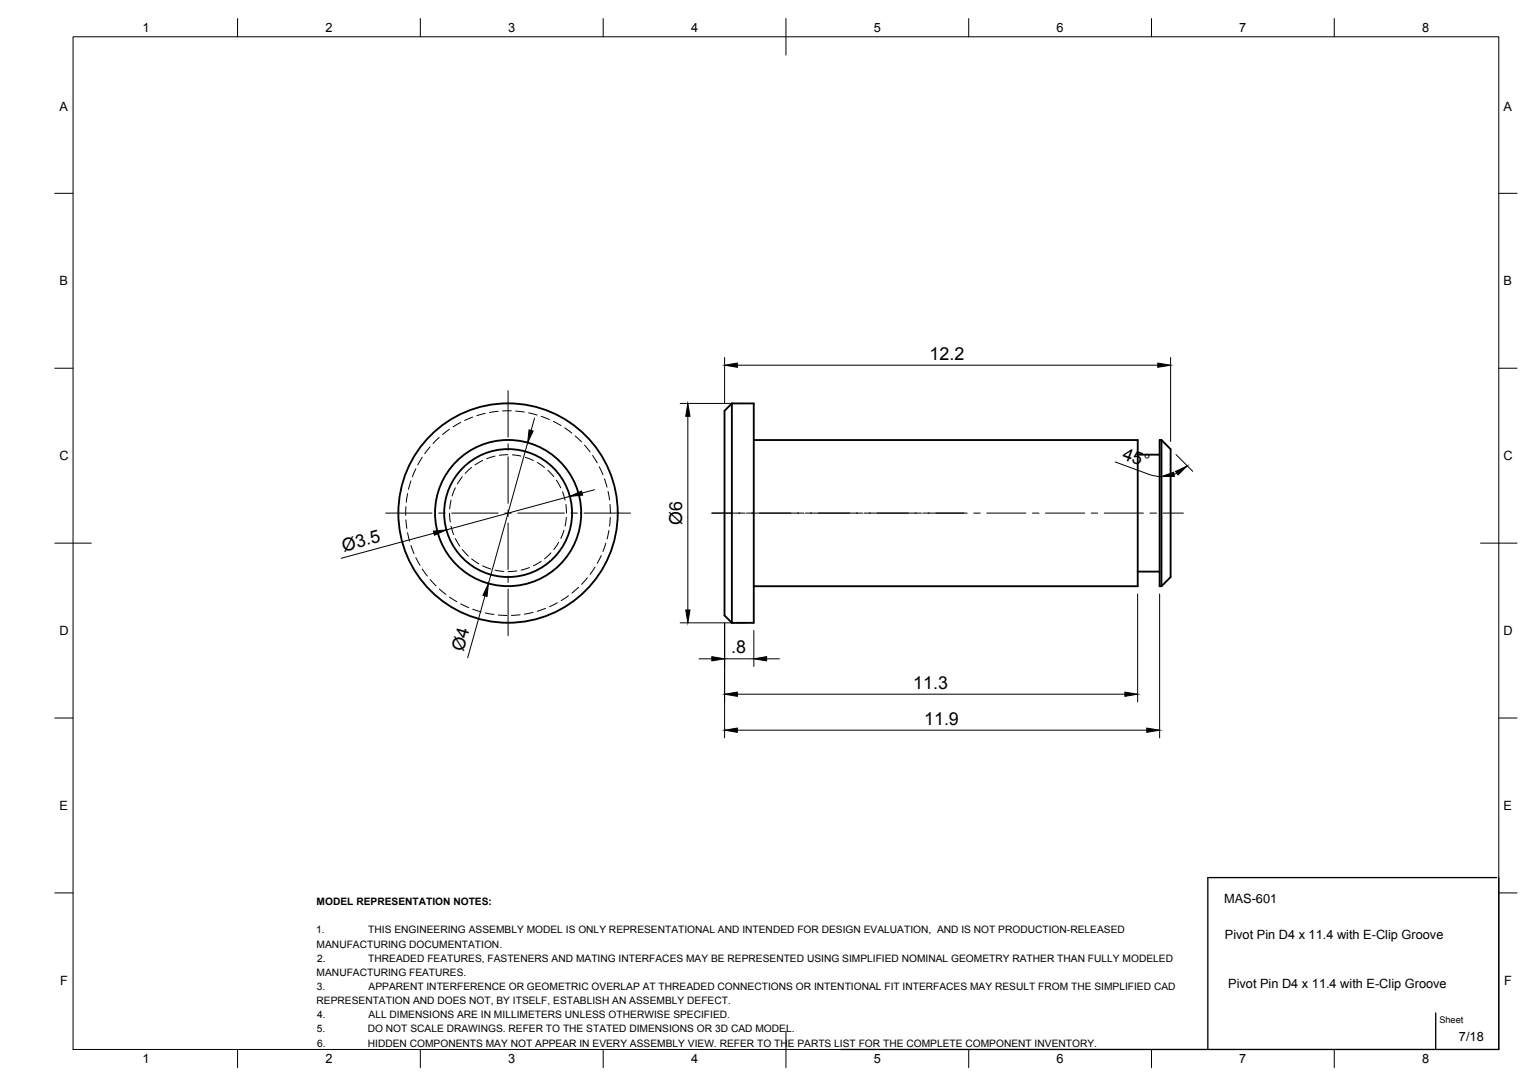
ISO-10303-21;
HEADER;
FILE_DESCRIPTION((''),'2;1');
FILE_NAME('Pivot Pin D4 x 11.4 with E-Clip Groove.step','2026-10-06T07:37:42+05:00',(''),(''),'','','');
FILE_SCHEMA (('AUTOMOTIVE_DESIGN { 1 0 10303 214 3 1 1 }'));
ENDSEC;
DATA;
#10=MECHANICAL_DESIGN_GEOMETRIC_PRESENTATION_REPRESENTATION('',(#383),#18757);
#349=SHAPE_REPRESENTATION_RELATIONSHIP('SRR','None',#18867,#366) ;
#366=ADVANCED_BREP_SHAPE_REPRESENTATION('',(#400),#18750) ;
#383=STYLED_ITEM('',(#18961),#400) ;
#400=MANIFOLD_SOLID_BREP('Pivot Pin D4 x 11.4 with E-Clip Groove',#9552) ;
#588=CYLINDRICAL_SURFACE('',#10224,3.) ;
#589=CYLINDRICAL_SURFACE('',#10228,2.) ;
#590=CYLINDRICAL_SURFACE('',#10232,1.59999999999999) ;
#591=CYLINDRICAL_SURFACE('',#10236,2.) ;
#729=FACE_BOUND('',#1946,.T.) ;
#730=FACE_BOUND('',#1949,.T.) ;
#731=FACE_BOUND('',#1952,.T.) ;
#906=PLANE('',#10220) ;
#907=PLANE('',#10226) ;
#908=PLANE('',#10230) ;
#909=PLANE('',#10234) ;
#910=PLANE('',#10240) ;
#1345=FACE_OUTER_BOUND('',#1942,.T.) ;
#1346=FACE_OUTER_BOUND('',#1943,.T.) ;
#1347=FACE_OUTER_BOUND('',#1944,.T.) ;
#1348=FACE_OUTER_BOUND('',#1945,.T.) ;
#1349=FACE_OUTER_BOUND('',#1947,.T.) ;
#1350=FACE_OUTER_BOUND('',#1948,.T.) ;
#1351=FACE_OUTER_BOUND('',#1950,.T.) ;
#1352=FACE_OUTER_BOUND('',#1951,.T.) ;
#1353=FACE_OUTER_BOUND('',#1953,.T.) ;
#1354=FACE_OUTER_BOUND('',#1954,.T.) ;
#1355=FACE_OUTER_BOUND('',#1955,.T.) ;
#1942=EDGE_LOOP('',(#7637)) ;
#1943=EDGE_LOOP('',(#7638,#7639,#7640,#7641)) ;
#1944=EDGE_LOOP('',(#7642,#7643,#7644,#7645)) ;
#1945=EDGE_LOOP('',(#7646)) ;
#1946=EDGE_LOOP('',(#7647)) ;
#1947=EDGE_LOOP('',(#7648,#7649,#7650,#7651)) ;
#1948=EDGE_LOOP('',(#7652)) ;
#1949=EDGE_LOOP('',(#7653)) ;
#1950=EDGE_LOOP('',(#7654,#7655,#7656,#7657)) ;
#1951=EDGE_LOOP('',(#7658)) ;
#1952=EDGE_LOOP('',(#7659)) ;
#1953=EDGE_LOOP('',(#7660,#7661,#7662,#7663)) ;
#1954=EDGE_LOOP('',(#7664,#7665,#7666,#7667)) ;
#1955=EDGE_LOOP('',(#7668)) ;
#2646=LINE('',#15200,#3417) ;
#2647=LINE('',#15204,#3418) ;
#2648=LINE('',#15211,#3419) ;
#2649=LINE('',#15218,#3420) ;
#2650=LINE('',#15225,#3421) ;
#2651=LINE('',#15229,#3422) ;
#3417=VECTOR('',#12082,2.9) ;
#3418=VECTOR('',#12087,3.) ;
#3419=VECTOR('',#12096,2.) ;
#3420=VECTOR('',#12105,1.59999999999999) ;
#3421=VECTOR('',#12114,2.) ;
#3422=VECTOR('',#12119,1.875) ;
#3978=CIRCLE('',#10221,2.79999999999999) ;
#3979=CIRCLE('',#10223,3.) ;
#3980=CIRCLE('',#10225,3.) ;
#3981=CIRCLE('',#10227,2.) ;
#3982=CIRCLE('',#10229,2.) ;
#3983=CIRCLE('',#10231,1.59999999999999) ;
#3984=CIRCLE('',#10233,1.59999999999999) ;
#3985=CIRCLE('',#10235,2.) ;
#3986=CIRCLE('',#10237,2.) ;
#3987=CIRCLE('',#10239,1.75) ;
#4575=VERTEX_POINT('',#15195) ;
#4576=VERTEX_POINT('',#15198) ;
#4577=VERTEX_POINT('',#15202) ;
#4578=VERTEX_POINT('',#15206) ;
#4579=VERTEX_POINT('',#15209) ;
#4580=VERTEX_POINT('',#15213) ;
#4581=VERTEX_POINT('',#15216) ;
#4582=VERTEX_POINT('',#15220) ;
#4583=VERTEX_POINT('',#15223) ;
#4584=VERTEX_POINT('',#15227) ;
#5665=EDGE_CURVE('',#4575,#4575,#3978,.T.) ;
#5666=EDGE_CURVE('',#4576,#4576,#3979,.T.) ;
#5667=EDGE_CURVE('',#4576,#4575,#2646,.T.) ;
#5668=EDGE_CURVE('',#4577,#4577,#3980,.T.) ;
#5669=EDGE_CURVE('',#4577,#4576,#2647,.T.) ;
#5670=EDGE_CURVE('',#4578,#4578,#3981,.T.) ;
#5671=EDGE_CURVE('',#4579,#4579,#3982,.T.) ;
#5672=EDGE_CURVE('',#4579,#4578,#2648,.T.) ;
#5673=EDGE_CURVE('',#4580,#4580,#3983,.T.) ;
#5674=EDGE_CURVE('',#4581,#4581,#3984,.T.) ;
#5675=EDGE_CURVE('',#4581,#4580,#2649,.T.) ;
#5676=EDGE_CURVE('',#4582,#4582,#3985,.T.) ;
#5677=EDGE_CURVE('',#4583,#4583,#3986,.T.) ;
#5678=EDGE_CURVE('',#4583,#4582,#2650,.T.) ;
#5679=EDGE_CURVE('',#4584,#4584,#3987,.T.) ;
#5680=EDGE_CURVE('',#4584,#4583,#2651,.T.) ;
#7637=ORIENTED_EDGE('',*,*,#5665,.F.) ;
#7638=ORIENTED_EDGE('',*,*,#5666,.F.) ;
#7639=ORIENTED_EDGE('',*,*,#5667,.T.) ;
#7640=ORIENTED_EDGE('',*,*,#5665,.T.) ;
#7641=ORIENTED_EDGE('',*,*,#5667,.F.) ;
#7642=ORIENTED_EDGE('',*,*,#5668,.F.) ;
#7643=ORIENTED_EDGE('',*,*,#5669,.T.) ;
#7644=ORIENTED_EDGE('',*,*,#5666,.T.) ;
#7645=ORIENTED_EDGE('',*,*,#5669,.F.) ;
#7646=ORIENTED_EDGE('',*,*,#5668,.T.) ;
#7647=ORIENTED_EDGE('',*,*,#5670,.F.) ;
#7648=ORIENTED_EDGE('',*,*,#5671,.F.) ;
#7649=ORIENTED_EDGE('',*,*,#5672,.T.) ;
#7650=ORIENTED_EDGE('',*,*,#5670,.T.) ;
#7651=ORIENTED_EDGE('',*,*,#5672,.F.) ;
#7652=ORIENTED_EDGE('',*,*,#5671,.T.) ;
#7653=ORIENTED_EDGE('',*,*,#5673,.F.) ;
#7654=ORIENTED_EDGE('',*,*,#5674,.F.) ;
#7655=ORIENTED_EDGE('',*,*,#5675,.T.) ;
#7656=ORIENTED_EDGE('',*,*,#5673,.T.) ;
#7657=ORIENTED_EDGE('',*,*,#5675,.F.) ;
#7658=ORIENTED_EDGE('',*,*,#5676,.F.) ;
#7659=ORIENTED_EDGE('',*,*,#5674,.T.) ;
#7660=ORIENTED_EDGE('',*,*,#5677,.F.) ;
#7661=ORIENTED_EDGE('',*,*,#5678,.T.) ;
#7662=ORIENTED_EDGE('',*,*,#5676,.T.) ;
#7663=ORIENTED_EDGE('',*,*,#5678,.F.) ;
#7664=ORIENTED_EDGE('',*,*,#5679,.F.) ;
#7665=ORIENTED_EDGE('',*,*,#5680,.T.) ;
#7666=ORIENTED_EDGE('',*,*,#5677,.T.) ;
#7667=ORIENTED_EDGE('',*,*,#5680,.F.) ;
#7668=ORIENTED_EDGE('',*,*,#5679,.T.) ;
#9010=CONICAL_SURFACE('',#10222,2.9,0.78539816339747) ;
#9011=CONICAL_SURFACE('',#10238,1.875,0.785398163397448) ;
#9281=ADVANCED_FACE('',(#1345),#906,.T.) ;
#9282=ADVANCED_FACE('',(#1346),#9010,.T.) ;
#9283=ADVANCED_FACE('',(#1347),#588,.T.) ;
#9284=ADVANCED_FACE('',(#1348,#729),#907,.T.) ;
#9285=ADVANCED_FACE('',(#1349),#589,.T.) ;
#9286=ADVANCED_FACE('',(#1350,#730),#908,.T.) ;
#9287=ADVANCED_FACE('',(#1351),#590,.T.) ;
#9288=ADVANCED_FACE('',(#1352,#731),#909,.T.) ;
#9289=ADVANCED_FACE('',(#1353),#591,.T.) ;
#9290=ADVANCED_FACE('',(#1354),#9011,.T.) ;
#9291=ADVANCED_FACE('',(#1355),#910,.T.) ;
#9552=CLOSED_SHELL('',(#9281,#9282,#9283,#9284,#9285,#9286,#9287,#9288,
#9289,#9290,#9291)) ;
#10219=AXIS2_PLACEMENT_3D('',#15193,#12072,#12073) ;
#10220=AXIS2_PLACEMENT_3D('',#15194,#12074,#12075) ;
#10221=AXIS2_PLACEMENT_3D('',#15196,#12076,#12077) ;
#10222=AXIS2_PLACEMENT_3D('',#15197,#12078,#12079) ;
#10223=AXIS2_PLACEMENT_3D('',#15199,#12080,#12081) ;
#10224=AXIS2_PLACEMENT_3D('',#15201,#12083,#12084) ;
#10225=AXIS2_PLACEMENT_3D('',#15203,#12085,#12086) ;
#10226=AXIS2_PLACEMENT_3D('',#15205,#12088,#12089) ;
#10227=AXIS2_PLACEMENT_3D('',#15207,#12090,#12091) ;
#10228=AXIS2_PLACEMENT_3D('',#15208,#12092,#12093) ;
#10229=AXIS2_PLACEMENT_3D('',#15210,#12094,#12095) ;
#10230=AXIS2_PLACEMENT_3D('',#15212,#12097,#12098) ;
#10231=AXIS2_PLACEMENT_3D('',#15214,#12099,#12100) ;
#10232=AXIS2_PLACEMENT_3D('',#15215,#12101,#12102) ;
#10233=AXIS2_PLACEMENT_3D('',#15217,#12103,#12104) ;
#10234=AXIS2_PLACEMENT_3D('',#15219,#12106,#12107) ;
#10235=AXIS2_PLACEMENT_3D('',#15221,#12108,#12109) ;
#10236=AXIS2_PLACEMENT_3D('',#15222,#12110,#12111) ;
#10237=AXIS2_PLACEMENT_3D('',#15224,#12112,#12113) ;
#10238=AXIS2_PLACEMENT_3D('',#15226,#12115,#12116) ;
#10239=AXIS2_PLACEMENT_3D('',#15228,#12117,#12118) ;
#10240=AXIS2_PLACEMENT_3D('',#15230,#12120,#12121) ;
#12072=DIRECTION('axis',(0.,0.,1.)) ;
#12073=DIRECTION('refdir',(1.,0.,0.)) ;
#12074=DIRECTION('center_axis',(0.,1.,0.)) ;
#12075=DIRECTION('ref_axis',(0.,0.,1.)) ;
#12076=DIRECTION('center_axis',(0.,-1.,0.)) ;
#12077=DIRECTION('ref_axis',(1.,0.,0.)) ;
#12078=DIRECTION('center_axis',(0.,-1.,0.)) ;
#12079=DIRECTION('ref_axis',(1.,0.,0.)) ;
#12080=DIRECTION('center_axis',(0.,-1.,0.)) ;
#12081=DIRECTION('ref_axis',(1.,0.,0.)) ;
#12082=DIRECTION('',(0.707106781186563,0.707106781186532,8.65956056235513E-17)) ;
#12083=DIRECTION('center_axis',(0.,-1.,0.)) ;
#12084=DIRECTION('ref_axis',(1.,0.,0.)) ;
#12085=DIRECTION('center_axis',(0.,-1.,0.)) ;
#12086=DIRECTION('ref_axis',(1.,0.,0.)) ;
#12087=DIRECTION('',(0.,1.,0.)) ;
#12088=DIRECTION('center_axis',(0.,-1.,0.)) ;
#12089=DIRECTION('ref_axis',(0.,0.,-1.)) ;
#12090=DIRECTION('center_axis',(0.,-1.,0.)) ;
#12091=DIRECTION('ref_axis',(1.,0.,0.)) ;
#12092=DIRECTION('center_axis',(0.,-1.,0.)) ;
#12093=DIRECTION('ref_axis',(1.,0.,0.)) ;
#12094=DIRECTION('center_axis',(0.,-1.,0.)) ;
#12095=DIRECTION('ref_axis',(1.,0.,0.)) ;
#12096=DIRECTION('',(0.,1.,0.)) ;
#12097=DIRECTION('center_axis',(0.,-1.,0.)) ;
#12098=DIRECTION('ref_axis',(0.,0.,-1.)) ;
#12099=DIRECTION('center_axis',(0.,-1.,0.)) ;
#12100=DIRECTION('ref_axis',(1.,0.,0.)) ;
#12101=DIRECTION('center_axis',(0.,-1.,0.)) ;
#12102=DIRECTION('ref_axis',(1.,0.,0.)) ;
#12103=DIRECTION('center_axis',(0.,-1.,0.)) ;
#12104=DIRECTION('ref_axis',(1.,0.,0.)) ;
#12105=DIRECTION('',(0.,1.,0.)) ;
#12106=DIRECTION('center_axis',(0.,1.,0.)) ;
#12107=DIRECTION('ref_axis',(0.,0.,1.)) ;
#12108=DIRECTION('center_axis',(0.,-1.,0.)) ;
#12109=DIRECTION('ref_axis',(1.,0.,0.)) ;
#12110=DIRECTION('center_axis',(0.,-1.,0.)) ;
#12111=DIRECTION('ref_axis',(1.,0.,0.)) ;
#12112=DIRECTION('center_axis',(0.,-1.,0.)) ;
#12113=DIRECTION('ref_axis',(1.,0.,0.)) ;
#12114=DIRECTION('',(0.,1.,0.)) ;
#12115=DIRECTION('center_axis',(0.,1.,0.)) ;
#12116=DIRECTION('ref_axis',(1.,0.,0.)) ;
#12117=DIRECTION('center_axis',(0.,-1.,0.)) ;
#12118=DIRECTION('ref_axis',(1.,0.,0.)) ;
#12119=DIRECTION('',(-0.707106781186548,0.707106781186547,-8.65956056235493E-17)) ;
#12120=DIRECTION('center_axis',(0.,-1.,0.)) ;
#12121=DIRECTION('ref_axis',(0.,0.,-1.)) ;
#15193=CARTESIAN_POINT('',(0.,0.,0.)) ;
#15194=CARTESIAN_POINT('Origin',(74.8,56.1,35.)) ;
#15195=CARTESIAN_POINT('',(69.2,56.1,35.)) ;
#15196=CARTESIAN_POINT('Origin',(72.,56.1,35.)) ;
#15197=CARTESIAN_POINT('Origin',(72.,56.,35.)) ;
#15198=CARTESIAN_POINT('',(69.,55.9,35.)) ;
#15199=CARTESIAN_POINT('Origin',(72.,55.9,35.)) ;
#15200=CARTESIAN_POINT('',(69.1,56.,35.)) ;
#15201=CARTESIAN_POINT('Origin',(72.,55.6,35.)) ;
#15202=CARTESIAN_POINT('',(69.,55.3,35.)) ;
#15203=CARTESIAN_POINT('Origin',(72.,55.3,35.)) ;
#15204=CARTESIAN_POINT('',(69.,55.6,35.)) ;
#15205=CARTESIAN_POINT('Origin',(74.,55.3,35.)) ;
#15206=CARTESIAN_POINT('',(70.,55.3,35.)) ;
#15207=CARTESIAN_POINT('Origin',(72.,55.3,35.)) ;
#15208=CARTESIAN_POINT('Origin',(72.,50.05,35.)) ;
#15209=CARTESIAN_POINT('',(70.,44.8,35.)) ;
#15210=CARTESIAN_POINT('Origin',(72.,44.8,35.)) ;
#15211=CARTESIAN_POINT('',(70.,50.05,35.)) ;
#15212=CARTESIAN_POINT('Origin',(73.6,44.8,35.)) ;
#15213=CARTESIAN_POINT('',(70.4,44.8,35.)) ;
#15214=CARTESIAN_POINT('Origin',(72.,44.8,35.)) ;
#15215=CARTESIAN_POINT('Origin',(72.,44.5,35.)) ;
#15216=CARTESIAN_POINT('',(70.4,44.2,35.)) ;
#15217=CARTESIAN_POINT('Origin',(72.,44.2,35.)) ;
#15218=CARTESIAN_POINT('',(70.4,44.5,35.)) ;
#15219=CARTESIAN_POINT('Origin',(74.,44.2,35.)) ;
#15220=CARTESIAN_POINT('',(70.,44.2,35.)) ;
#15221=CARTESIAN_POINT('Origin',(72.,44.2,35.)) ;
#15222=CARTESIAN_POINT('Origin',(72.,44.175,35.)) ;
#15223=CARTESIAN_POINT('',(70.,44.15,35.)) ;
#15224=CARTESIAN_POINT('Origin',(72.,44.15,35.)) ;
#15225=CARTESIAN_POINT('',(70.,44.175,35.)) ;
#15226=CARTESIAN_POINT('Origin',(72.,44.025,35.)) ;
#15227=CARTESIAN_POINT('',(70.25,43.9,35.)) ;
#15228=CARTESIAN_POINT('Origin',(72.,43.9,35.)) ;
#15229=CARTESIAN_POINT('',(70.125,44.025,35.)) ;
#15230=CARTESIAN_POINT('Origin',(72.,43.9,35.)) ;
#18731=UNCERTAINTY_MEASURE_WITH_UNIT(LENGTH_MEASURE(0.01),#18758,
'DISTANCE_ACCURACY_VALUE',
'Maximum model space distance between geometric entities at asserted c
onnectivities') ;
#18738=UNCERTAINTY_MEASURE_WITH_UNIT(LENGTH_MEASURE(0.01),#18758,
'DISTANCE_ACCURACY_VALUE',
'Maximum model space distance between geometric entities at asserted c
onnectivities') ;
#18750=(
GEOMETRIC_REPRESENTATION_CONTEXT(3)
GLOBAL_UNCERTAINTY_ASSIGNED_CONTEXT((#18731))
GLOBAL_UNIT_ASSIGNED_CONTEXT((#18758,#18760,#18761))
REPRESENTATION_CONTEXT('','3D')
) ;
#18757=(
GEOMETRIC_REPRESENTATION_CONTEXT(3)
GLOBAL_UNCERTAINTY_ASSIGNED_CONTEXT((#18738))
GLOBAL_UNIT_ASSIGNED_CONTEXT((#18758,#18760,#18761))
REPRESENTATION_CONTEXT('','3D')
) ;
#18758=(
LENGTH_UNIT()
NAMED_UNIT(*)
SI_UNIT(.MILLI.,.METRE.)
) ;
#18760=(
NAMED_UNIT(*)
PLANE_ANGLE_UNIT()
SI_UNIT($,.RADIAN.)
) ;
#18761=(
NAMED_UNIT(*)
SI_UNIT($,.STERADIAN.)
SOLID_ANGLE_UNIT()
) ;
#18773=SHAPE_DEFINITION_REPRESENTATION(#18791,#18867) ;
#18791=PRODUCT_DEFINITION_SHAPE('',$,#18886) ;
#18867=SHAPE_REPRESENTATION('',(#10219),#18750) ;
#18874=PRODUCT_DEFINITION_CONTEXT('part definition',#18930,'design') ;
#18886=PRODUCT_DEFINITION('Pivot Pin D4 x 11.4 with E-Clip Groove',
'Pivot Pin D4 x 11.4 with E-Clip Groove',#18904,#18874) ;
#18904=PRODUCT_DEFINITION_FORMATION('',$,#18943) ;
#18930=APPLICATION_CONTEXT(
'Core Data for Automotive Mechanical Design Process') ;
#18931=PRODUCT_CONTEXT('part definition',#18930,'mechanical') ;
#18943=PRODUCT('Pivot Pin D4 x 11.4 with E-Clip Groove',
'Pivot Pin D4 x 11.4 with E-Clip Groove',$,(#18931)) ;
#18961=PRESENTATION_STYLE_ASSIGNMENT((#18979)) ;
#18979=SURFACE_STYLE_USAGE(.BOTH.,#18997) ;
#18997=SURFACE_SIDE_STYLE('',(#19015)) ;
#19015=SURFACE_STYLE_FILL_AREA(#19033) ;
#19033=FILL_AREA_STYLE(
'MAS-253 Metallic Sheet - Pivot Pin D4 x 11.4 with E-Clip Groove',(#19051)) ;
#19051=FILL_AREA_STYLE_COLOUR(
'MAS-253 Metallic Sheet - Pivot Pin D4 x 11.4 with E-Clip Groove',#19069) ;
#19069=COLOUR_RGB(
'MAS-253 Metallic Sheet - Pivot Pin D4 x 11.4 with E-Clip Groove', 0.08235294, 0.09019608, 0.10196078) ;
ENDSEC;
END-ISO-10303-21;
